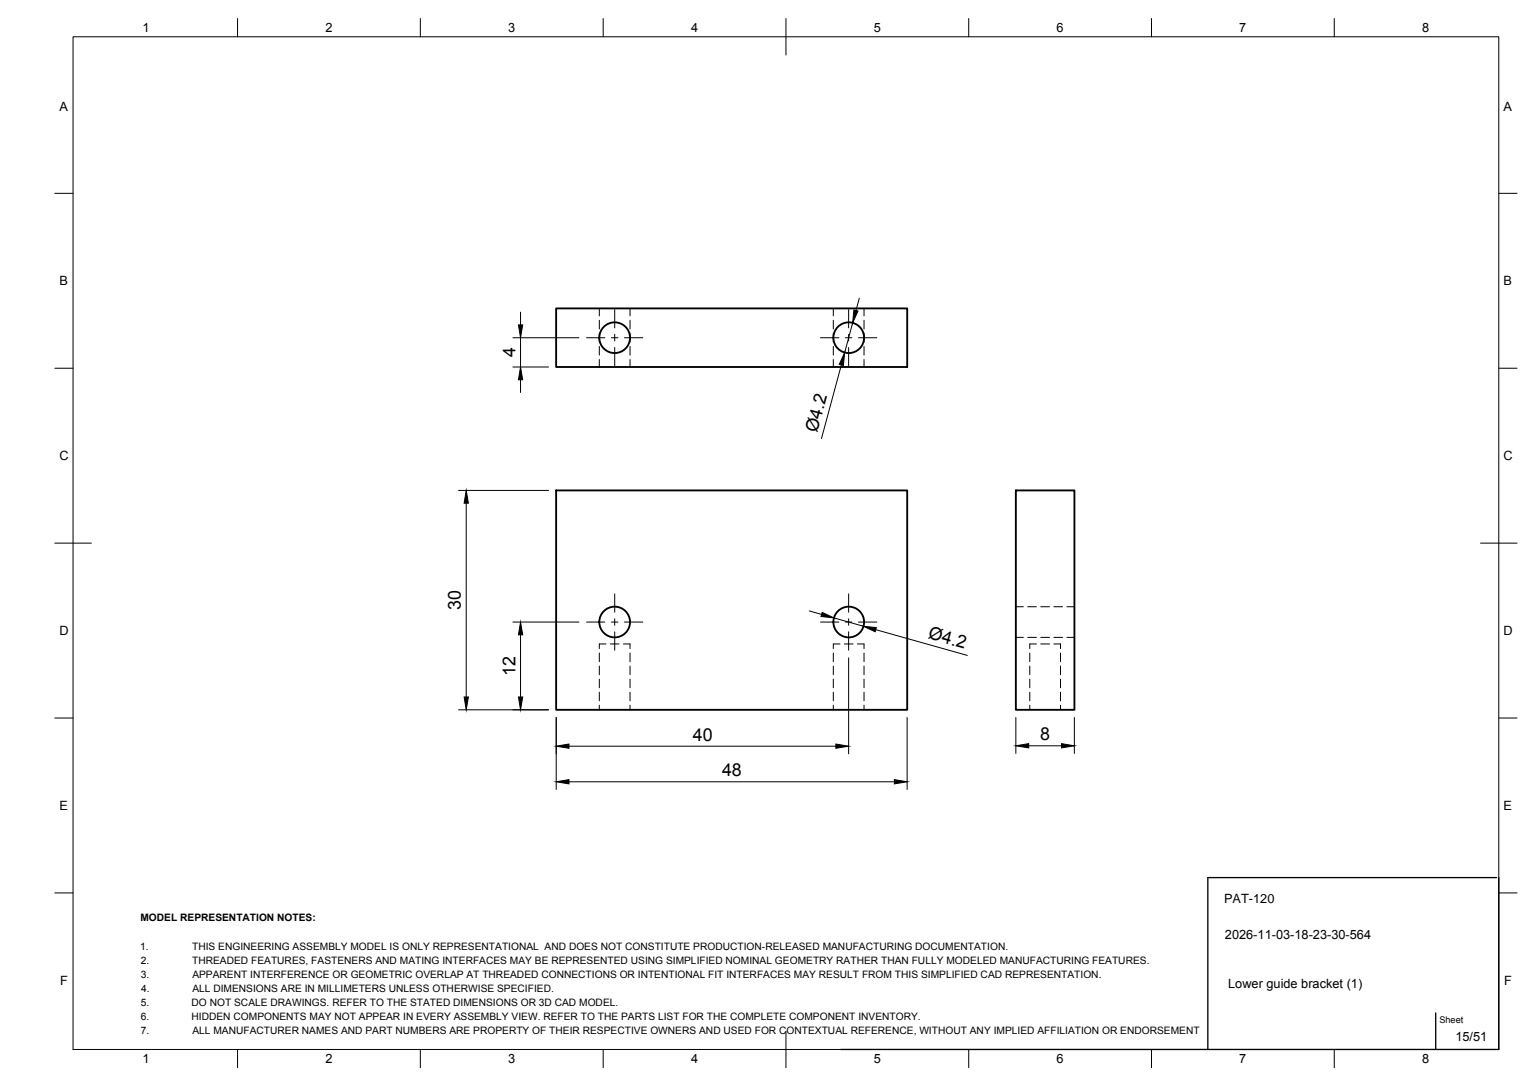
ISO-10303-21;
HEADER;
/* Generated by software containing ST-Developer
 * from STEP Tools, Inc. (www.steptools.com) 
 */

FILE_DESCRIPTION(
/* description */ ('Vibration shaker table dummy'),
/* implementation_level */ '2;1');

FILE_NAME(
/* name */ 'Lower guide bracket (1).step',
/* time_stamp */ '2026-10-27T10:55:14-07:00',
/* author */ (''),
/* organization */ (''),
/* preprocessor_version */ 'ST-DEVELOPER v20.2',
/* originating_system */ 'Autodesk Translation Framework v15.17.0.0',
/* authorisation */ '');

FILE_SCHEMA (('AUTOMOTIVE_DESIGN { 1 0 10303 214 3 1 1 }'));
ENDSEC;

DATA;
#10=MECHANICAL_DESIGN_GEOMETRIC_PRESENTATION_REPRESENTATION('',(#696),#22394);
#604=SHAPE_REPRESENTATION_RELATIONSHIP('SRR','None',#22650,#650);
#650=ADVANCED_BREP_SHAPE_REPRESENTATION('',(#742),#22356);
#696=STYLED_ITEM('',(#22940),#742);
#742=MANIFOLD_SOLID_BREP('Body1',#9214);
#877=FACE_BOUND('',#2073,.T.);
#878=FACE_BOUND('',#2074,.T.);
#879=FACE_BOUND('',#2077,.T.);
#880=FACE_BOUND('',#2078,.T.);
#881=FACE_BOUND('',#2082,.T.);
#882=FACE_BOUND('',#2083,.T.);
#1126=PLANE('',#10022);
#1127=PLANE('',#10026);
#1128=PLANE('',#10033);
#1129=PLANE('',#10034);
#1130=PLANE('',#10035);
#1131=PLANE('',#10036);
#1132=PLANE('',#10037);
#1133=PLANE('',#10038);
#1466=FACE_OUTER_BOUND('',#2066,.T.);
#1467=FACE_OUTER_BOUND('',#2067,.T.);
#1468=FACE_OUTER_BOUND('',#2068,.T.);
#1469=FACE_OUTER_BOUND('',#2069,.T.);
#1470=FACE_OUTER_BOUND('',#2070,.T.);
#1471=FACE_OUTER_BOUND('',#2071,.T.);
#1472=FACE_OUTER_BOUND('',#2072,.T.);
#1473=FACE_OUTER_BOUND('',#2075,.T.);
#1474=FACE_OUTER_BOUND('',#2076,.T.);
#1475=FACE_OUTER_BOUND('',#2079,.T.);
#1476=FACE_OUTER_BOUND('',#2080,.T.);
#1477=FACE_OUTER_BOUND('',#2081,.T.);
#2066=EDGE_LOOP('',(#6828,#6829,#6830,#6831));
#2067=EDGE_LOOP('',(#6832));
#2068=EDGE_LOOP('',(#6833,#6834,#6835,#6836));
#2069=EDGE_LOOP('',(#6837));
#2070=EDGE_LOOP('',(#6838,#6839,#6840,#6841));
#2071=EDGE_LOOP('',(#6842,#6843,#6844,#6845));
#2072=EDGE_LOOP('',(#6846,#6847,#6848,#6849));
#2073=EDGE_LOOP('',(#6850));
#2074=EDGE_LOOP('',(#6851));
#2075=EDGE_LOOP('',(#6852,#6853,#6854,#6855));
#2076=EDGE_LOOP('',(#6856,#6857,#6858,#6859));
#2077=EDGE_LOOP('',(#6860));
#2078=EDGE_LOOP('',(#6861));
#2079=EDGE_LOOP('',(#6862,#6863,#6864,#6865));
#2080=EDGE_LOOP('',(#6866,#6867,#6868,#6869));
#2081=EDGE_LOOP('',(#6870,#6871,#6872,#6873));
#2082=EDGE_LOOP('',(#6874));
#2083=EDGE_LOOP('',(#6875));
#2790=LINE('',#16048,#3409);
#2791=LINE('',#16055,#3410);
#2792=LINE('',#16062,#3411);
#2793=LINE('',#16068,#3412);
#2794=LINE('',#16073,#3413);
#2795=LINE('',#16075,#3414);
#2796=LINE('',#16077,#3415);
#2797=LINE('',#16078,#3416);
#2798=LINE('',#16081,#3417);
#2799=LINE('',#16083,#3418);
#2800=LINE('',#16084,#3419);
#2801=LINE('',#16087,#3420);
#2802=LINE('',#16089,#3421);
#2803=LINE('',#16090,#3422);
#2804=LINE('',#16092,#3423);
#2805=LINE('',#16093,#3424);
#3409=VECTOR('',#11640,0.21);
#3410=VECTOR('',#11649,0.21);
#3411=VECTOR('',#11658,0.21);
#3412=VECTOR('',#11665,0.21);
#3413=VECTOR('',#11670,1.);
#3414=VECTOR('',#11671,1.);
#3415=VECTOR('',#11672,1.);
#3416=VECTOR('',#11673,1.);
#3417=VECTOR('',#11676,1.);
#3418=VECTOR('',#11677,1.);
#3419=VECTOR('',#11678,1.);
#3420=VECTOR('',#11681,1.);
#3421=VECTOR('',#11682,1.);
#3422=VECTOR('',#11683,1.);
#3423=VECTOR('',#11686,1.);
#3424=VECTOR('',#11687,1.);
#3982=CIRCLE('',#10020,0.21);
#3983=CIRCLE('',#10021,0.21);
#3984=CIRCLE('',#10024,0.21);
#3985=CIRCLE('',#10025,0.21);
#3986=CIRCLE('',#10028,0.21);
#3987=CIRCLE('',#10029,0.21);
#3988=CIRCLE('',#10031,0.21);
#3989=CIRCLE('',#10032,0.21);
#4561=VERTEX_POINT('',#16045);
#4562=VERTEX_POINT('',#16047);
#4563=VERTEX_POINT('',#16052);
#4564=VERTEX_POINT('',#16054);
#4565=VERTEX_POINT('',#16059);
#4566=VERTEX_POINT('',#16061);
#4567=VERTEX_POINT('',#16065);
#4568=VERTEX_POINT('',#16067);
#4569=VERTEX_POINT('',#16071);
#4570=VERTEX_POINT('',#16072);
#4571=VERTEX_POINT('',#16074);
#4572=VERTEX_POINT('',#16076);
#4573=VERTEX_POINT('',#16080);
#4574=VERTEX_POINT('',#16082);
#4575=VERTEX_POINT('',#16086);
#4576=VERTEX_POINT('',#16088);
#5407=EDGE_CURVE('',#4561,#4561,#3982,.T.);
#5408=EDGE_CURVE('',#4561,#4562,#2790,.T.);
#5409=EDGE_CURVE('',#4562,#4562,#3983,.T.);
#5410=EDGE_CURVE('',#4563,#4563,#3984,.T.);
#5411=EDGE_CURVE('',#4563,#4564,#2791,.T.);
#5412=EDGE_CURVE('',#4564,#4564,#3985,.T.);
#5413=EDGE_CURVE('',#4565,#4565,#3986,.T.);
#5414=EDGE_CURVE('',#4565,#4566,#2792,.T.);
#5415=EDGE_CURVE('',#4566,#4566,#3987,.T.);
#5416=EDGE_CURVE('',#4567,#4567,#3988,.T.);
#5417=EDGE_CURVE('',#4567,#4568,#2793,.T.);
#5418=EDGE_CURVE('',#4568,#4568,#3989,.T.);
#5419=EDGE_CURVE('',#4569,#4570,#2794,.T.);
#5420=EDGE_CURVE('',#4570,#4571,#2795,.T.);
#5421=EDGE_CURVE('',#4572,#4571,#2796,.T.);
#5422=EDGE_CURVE('',#4569,#4572,#2797,.T.);
#5423=EDGE_CURVE('',#4573,#4569,#2798,.T.);
#5424=EDGE_CURVE('',#4574,#4572,#2799,.T.);
#5425=EDGE_CURVE('',#4573,#4574,#2800,.T.);
#5426=EDGE_CURVE('',#4575,#4573,#2801,.T.);
#5427=EDGE_CURVE('',#4576,#4574,#2802,.T.);
#5428=EDGE_CURVE('',#4575,#4576,#2803,.T.);
#5429=EDGE_CURVE('',#4570,#4575,#2804,.T.);
#5430=EDGE_CURVE('',#4571,#4576,#2805,.T.);
#6828=ORIENTED_EDGE('',*,*,#5407,.F.);
#6829=ORIENTED_EDGE('',*,*,#5408,.T.);
#6830=ORIENTED_EDGE('',*,*,#5409,.T.);
#6831=ORIENTED_EDGE('',*,*,#5408,.F.);
#6832=ORIENTED_EDGE('',*,*,#5409,.F.);
#6833=ORIENTED_EDGE('',*,*,#5410,.F.);
#6834=ORIENTED_EDGE('',*,*,#5411,.T.);
#6835=ORIENTED_EDGE('',*,*,#5412,.T.);
#6836=ORIENTED_EDGE('',*,*,#5411,.F.);
#6837=ORIENTED_EDGE('',*,*,#5412,.F.);
#6838=ORIENTED_EDGE('',*,*,#5413,.F.);
#6839=ORIENTED_EDGE('',*,*,#5414,.T.);
#6840=ORIENTED_EDGE('',*,*,#5415,.F.);
#6841=ORIENTED_EDGE('',*,*,#5414,.F.);
#6842=ORIENTED_EDGE('',*,*,#5416,.F.);
#6843=ORIENTED_EDGE('',*,*,#5417,.T.);
#6844=ORIENTED_EDGE('',*,*,#5418,.F.);
#6845=ORIENTED_EDGE('',*,*,#5417,.F.);
#6846=ORIENTED_EDGE('',*,*,#5419,.T.);
#6847=ORIENTED_EDGE('',*,*,#5420,.T.);
#6848=ORIENTED_EDGE('',*,*,#5421,.F.);
#6849=ORIENTED_EDGE('',*,*,#5422,.F.);
#6850=ORIENTED_EDGE('',*,*,#5415,.T.);
#6851=ORIENTED_EDGE('',*,*,#5418,.T.);
#6852=ORIENTED_EDGE('',*,*,#5423,.T.);
#6853=ORIENTED_EDGE('',*,*,#5422,.T.);
#6854=ORIENTED_EDGE('',*,*,#5424,.F.);
#6855=ORIENTED_EDGE('',*,*,#5425,.F.);
#6856=ORIENTED_EDGE('',*,*,#5426,.T.);
#6857=ORIENTED_EDGE('',*,*,#5425,.T.);
#6858=ORIENTED_EDGE('',*,*,#5427,.F.);
#6859=ORIENTED_EDGE('',*,*,#5428,.F.);
#6860=ORIENTED_EDGE('',*,*,#5413,.T.);
#6861=ORIENTED_EDGE('',*,*,#5416,.T.);
#6862=ORIENTED_EDGE('',*,*,#5429,.T.);
#6863=ORIENTED_EDGE('',*,*,#5428,.T.);
#6864=ORIENTED_EDGE('',*,*,#5430,.F.);
#6865=ORIENTED_EDGE('',*,*,#5420,.F.);
#6866=ORIENTED_EDGE('',*,*,#5430,.T.);
#6867=ORIENTED_EDGE('',*,*,#5427,.T.);
#6868=ORIENTED_EDGE('',*,*,#5424,.T.);
#6869=ORIENTED_EDGE('',*,*,#5421,.T.);
#6870=ORIENTED_EDGE('',*,*,#5429,.F.);
#6871=ORIENTED_EDGE('',*,*,#5419,.F.);
#6872=ORIENTED_EDGE('',*,*,#5423,.F.);
#6873=ORIENTED_EDGE('',*,*,#5426,.F.);
#6874=ORIENTED_EDGE('',*,*,#5407,.T.);
#6875=ORIENTED_EDGE('',*,*,#5410,.T.);
#8564=CYLINDRICAL_SURFACE('',#10019,0.21);
#8565=CYLINDRICAL_SURFACE('',#10023,0.21);
#8566=CYLINDRICAL_SURFACE('',#10027,0.21);
#8567=CYLINDRICAL_SURFACE('',#10030,0.21);
#8831=ADVANCED_FACE('',(#1466),#8564,.F.);
#8832=ADVANCED_FACE('',(#1467),#1126,.F.);
#8833=ADVANCED_FACE('',(#1468),#8565,.F.);
#8834=ADVANCED_FACE('',(#1469),#1127,.F.);
#8835=ADVANCED_FACE('',(#1470),#8566,.F.);
#8836=ADVANCED_FACE('',(#1471),#8567,.F.);
#8837=ADVANCED_FACE('',(#1472,#877,#878),#1128,.T.);
#8838=ADVANCED_FACE('',(#1473),#1129,.T.);
#8839=ADVANCED_FACE('',(#1474,#879,#880),#1130,.T.);
#8840=ADVANCED_FACE('',(#1475),#1131,.T.);
#8841=ADVANCED_FACE('',(#1476),#1132,.T.);
#8842=ADVANCED_FACE('',(#1477,#881,#882),#1133,.F.);
#9214=CLOSED_SHELL('',(#8831,#8832,#8833,#8834,#8835,#8836,#8837,#8838,
#8839,#8840,#8841,#8842));
#10018=AXIS2_PLACEMENT_3D('',#16043,#11634,#11635);
#10019=AXIS2_PLACEMENT_3D('',#16044,#11636,#11637);
#10020=AXIS2_PLACEMENT_3D('',#16046,#11638,#11639);
#10021=AXIS2_PLACEMENT_3D('',#16049,#11641,#11642);
#10022=AXIS2_PLACEMENT_3D('',#16050,#11643,#11644);
#10023=AXIS2_PLACEMENT_3D('',#16051,#11645,#11646);
#10024=AXIS2_PLACEMENT_3D('',#16053,#11647,#11648);
#10025=AXIS2_PLACEMENT_3D('',#16056,#11650,#11651);
#10026=AXIS2_PLACEMENT_3D('',#16057,#11652,#11653);
#10027=AXIS2_PLACEMENT_3D('',#16058,#11654,#11655);
#10028=AXIS2_PLACEMENT_3D('',#16060,#11656,#11657);
#10029=AXIS2_PLACEMENT_3D('',#16063,#11659,#11660);
#10030=AXIS2_PLACEMENT_3D('',#16064,#11661,#11662);
#10031=AXIS2_PLACEMENT_3D('',#16066,#11663,#11664);
#10032=AXIS2_PLACEMENT_3D('',#16069,#11666,#11667);
#10033=AXIS2_PLACEMENT_3D('',#16070,#11668,#11669);
#10034=AXIS2_PLACEMENT_3D('',#16079,#11674,#11675);
#10035=AXIS2_PLACEMENT_3D('',#16085,#11679,#11680);
#10036=AXIS2_PLACEMENT_3D('',#16091,#11684,#11685);
#10037=AXIS2_PLACEMENT_3D('',#16094,#11688,#11689);
#10038=AXIS2_PLACEMENT_3D('',#16095,#11690,#11691);
#11634=DIRECTION('axis',(0.,0.,1.));
#11635=DIRECTION('refdir',(1.,0.,0.));
#11636=DIRECTION('center_axis',(0.,0.,1.));
#11637=DIRECTION('ref_axis',(1.,0.,0.));
#11638=DIRECTION('center_axis',(0.,0.,1.));
#11639=DIRECTION('ref_axis',(1.,0.,0.));
#11640=DIRECTION('',(0.,0.,1.));
#11641=DIRECTION('center_axis',(0.,0.,1.));
#11642=DIRECTION('ref_axis',(1.,0.,0.));
#11643=DIRECTION('center_axis',(0.,0.,1.));
#11644=DIRECTION('ref_axis',(1.,0.,0.));
#11645=DIRECTION('center_axis',(0.,0.,1.));
#11646=DIRECTION('ref_axis',(1.,0.,0.));
#11647=DIRECTION('center_axis',(0.,0.,1.));
#11648=DIRECTION('ref_axis',(1.,0.,0.));
#11649=DIRECTION('',(0.,0.,1.));
#11650=DIRECTION('center_axis',(0.,0.,1.));
#11651=DIRECTION('ref_axis',(1.,0.,0.));
#11652=DIRECTION('center_axis',(0.,0.,1.));
#11653=DIRECTION('ref_axis',(1.,0.,0.));
#11654=DIRECTION('center_axis',(0.,1.,0.));
#11655=DIRECTION('ref_axis',(1.,0.,0.));
#11656=DIRECTION('center_axis',(0.,1.,0.));
#11657=DIRECTION('ref_axis',(1.,0.,0.));
#11658=DIRECTION('',(0.,1.,0.));
#11659=DIRECTION('center_axis',(0.,-1.,0.));
#11660=DIRECTION('ref_axis',(1.,0.,0.));
#11661=DIRECTION('center_axis',(0.,1.,0.));
#11662=DIRECTION('ref_axis',(1.,0.,0.));
#11663=DIRECTION('center_axis',(0.,1.,0.));
#11664=DIRECTION('ref_axis',(1.,0.,0.));
#11665=DIRECTION('',(0.,1.,0.));
#11666=DIRECTION('center_axis',(0.,-1.,0.));
#11667=DIRECTION('ref_axis',(1.,0.,0.));
#11668=DIRECTION('center_axis',(0.,1.,0.));
#11669=DIRECTION('ref_axis',(-1.,0.,0.));
#11670=DIRECTION('',(-1.,0.,0.));
#11671=DIRECTION('',(0.,0.,1.));
#11672=DIRECTION('',(-1.,0.,0.));
#11673=DIRECTION('',(0.,0.,1.));
#11674=DIRECTION('center_axis',(1.,0.,0.));
#11675=DIRECTION('ref_axis',(0.,1.,0.));
#11676=DIRECTION('',(0.,1.,0.));
#11677=DIRECTION('',(0.,1.,0.));
#11678=DIRECTION('',(0.,0.,1.));
#11679=DIRECTION('center_axis',(0.,-1.,0.));
#11680=DIRECTION('ref_axis',(1.,0.,0.));
#11681=DIRECTION('',(1.,0.,0.));
#11682=DIRECTION('',(1.,0.,0.));
#11683=DIRECTION('',(0.,0.,1.));
#11684=DIRECTION('center_axis',(-1.,0.,0.));
#11685=DIRECTION('ref_axis',(0.,-1.,0.));
#11686=DIRECTION('',(0.,-1.,0.));
#11687=DIRECTION('',(0.,-1.,0.));
#11688=DIRECTION('center_axis',(0.,0.,1.));
#11689=DIRECTION('ref_axis',(1.,0.,0.));
#11690=DIRECTION('center_axis',(0.,0.,1.));
#11691=DIRECTION('ref_axis',(1.,0.,0.));
#16043=CARTESIAN_POINT('',(0.,0.,0.));
#16044=CARTESIAN_POINT('Origin',(-7.6,6.7,-0.1));
#16045=CARTESIAN_POINT('',(-7.81,6.7,0.));
#16046=CARTESIAN_POINT('Origin',(-7.6,6.7,0.));
#16047=CARTESIAN_POINT('',(-7.81,6.7,0.9));
#16048=CARTESIAN_POINT('',(-7.81,6.7,-0.1));
#16049=CARTESIAN_POINT('Origin',(-7.6,6.7,0.9));
#16050=CARTESIAN_POINT('Origin',(-7.6,6.7,0.9));
#16051=CARTESIAN_POINT('Origin',(-4.4,6.7,-0.1));
#16052=CARTESIAN_POINT('',(-4.61,6.7,0.));
#16053=CARTESIAN_POINT('Origin',(-4.4,6.7,0.));
#16054=CARTESIAN_POINT('',(-4.61,6.7,0.9));
#16055=CARTESIAN_POINT('',(-4.61,6.7,-0.1));
#16056=CARTESIAN_POINT('Origin',(-4.4,6.7,0.9));
#16057=CARTESIAN_POINT('Origin',(-4.4,6.7,0.9));
#16058=CARTESIAN_POINT('Origin',(-7.6,6.2,1.2));
#16059=CARTESIAN_POINT('',(-7.81,6.3,1.2));
#16060=CARTESIAN_POINT('Origin',(-7.6,6.3,1.2));
#16061=CARTESIAN_POINT('',(-7.81,7.1,1.2));
#16062=CARTESIAN_POINT('',(-7.81,6.2,1.2));
#16063=CARTESIAN_POINT('Origin',(-7.6,7.1,1.2));
#16064=CARTESIAN_POINT('Origin',(-4.4,6.2,1.2));
#16065=CARTESIAN_POINT('',(-4.61,6.3,1.2));
#16066=CARTESIAN_POINT('Origin',(-4.4,6.3,1.2));
#16067=CARTESIAN_POINT('',(-4.61,7.1,1.2));
#16068=CARTESIAN_POINT('',(-4.61,6.2,1.2));
#16069=CARTESIAN_POINT('Origin',(-4.4,7.1,1.2));
#16070=CARTESIAN_POINT('Origin',(-3.6,7.1,0.));
#16071=CARTESIAN_POINT('',(-3.6,7.1,0.));
#16072=CARTESIAN_POINT('',(-8.4,7.1,0.));
#16073=CARTESIAN_POINT('',(-3.6,7.1,0.));
#16074=CARTESIAN_POINT('',(-8.4,7.1,3.));
#16075=CARTESIAN_POINT('',(-8.4,7.1,0.));
#16076=CARTESIAN_POINT('',(-3.6,7.1,3.));
#16077=CARTESIAN_POINT('',(-3.6,7.1,3.));
#16078=CARTESIAN_POINT('',(-3.6,7.1,0.));
#16079=CARTESIAN_POINT('Origin',(-3.6,6.3,0.));
#16080=CARTESIAN_POINT('',(-3.6,6.3,0.));
#16081=CARTESIAN_POINT('',(-3.6,6.3,0.));
#16082=CARTESIAN_POINT('',(-3.6,6.3,3.));
#16083=CARTESIAN_POINT('',(-3.6,6.3,3.));
#16084=CARTESIAN_POINT('',(-3.6,6.3,0.));
#16085=CARTESIAN_POINT('Origin',(-8.4,6.3,0.));
#16086=CARTESIAN_POINT('',(-8.4,6.3,0.));
#16087=CARTESIAN_POINT('',(-8.4,6.3,0.));
#16088=CARTESIAN_POINT('',(-8.4,6.3,3.));
#16089=CARTESIAN_POINT('',(-8.4,6.3,3.));
#16090=CARTESIAN_POINT('',(-8.4,6.3,0.));
#16091=CARTESIAN_POINT('Origin',(-8.4,7.1,0.));
#16092=CARTESIAN_POINT('',(-8.4,7.1,0.));
#16093=CARTESIAN_POINT('',(-8.4,7.1,3.));
#16094=CARTESIAN_POINT('Origin',(-6.,6.7,3.));
#16095=CARTESIAN_POINT('Origin',(-6.,6.7,0.));
#22305=UNCERTAINTY_MEASURE_WITH_UNIT(LENGTH_MEASURE(0.001),#22395,
'DISTANCE_ACCURACY_VALUE',
'Maximum model space distance between geometric entities at asserted c
onnectivities');
#22343=UNCERTAINTY_MEASURE_WITH_UNIT(LENGTH_MEASURE(0.001),#22395,
'DISTANCE_ACCURACY_VALUE',
'Maximum model space distance between geometric entities at asserted c
onnectivities');
#22356=(
GEOMETRIC_REPRESENTATION_CONTEXT(3)
GLOBAL_UNCERTAINTY_ASSIGNED_CONTEXT((#22305))
GLOBAL_UNIT_ASSIGNED_CONTEXT((#22395,#22397,#22398))
REPRESENTATION_CONTEXT('','3D')
);
#22394=(
GEOMETRIC_REPRESENTATION_CONTEXT(3)
GLOBAL_UNCERTAINTY_ASSIGNED_CONTEXT((#22343))
GLOBAL_UNIT_ASSIGNED_CONTEXT((#22395,#22397,#22398))
REPRESENTATION_CONTEXT('','3D')
);
#22395=(
LENGTH_UNIT()
NAMED_UNIT(*)
SI_UNIT(.CENTI.,.METRE.)
);
#22397=(
NAMED_UNIT(*)
PLANE_ANGLE_UNIT()
SI_UNIT($,.RADIAN.)
);
#22398=(
NAMED_UNIT(*)
SI_UNIT($,.STERADIAN.)
SOLID_ANGLE_UNIT()
);
#22411=SHAPE_DEFINITION_REPRESENTATION(#22461,#22650);
#22461=PRODUCT_DEFINITION_SHAPE('',$,#22701);
#22650=SHAPE_REPRESENTATION('',(#10018),#22356);
#22688=PRODUCT_DEFINITION_CONTEXT('part definition',#22840,'design');
#22701=PRODUCT_DEFINITION('Lower guide bracket (1)',
'Lower guide bracket (1)',#22751,#22688);
#22751=PRODUCT_DEFINITION_FORMATION('',$,#22854);
#22840=APPLICATION_CONTEXT(
'Core Data for Automotive Mechanical Design Process');
#22841=PRODUCT_CONTEXT('part definition',#22840,'mechanical');
#22854=PRODUCT('Lower guide bracket (1)','Lower guide bracket (1)',
'Lower guide bracket (1)',(#22841));
#22934=COLOUR_RGB('Dark Blue',0.08,0.2,0.34);
#22935=FILL_AREA_STYLE_COLOUR('',#22934);
#22936=FILL_AREA_STYLE('',(#22935));
#22937=SURFACE_STYLE_FILL_AREA(#22936);
#22938=SURFACE_SIDE_STYLE('',(#22937));
#22939=SURFACE_STYLE_USAGE(.BOTH.,#22938);
#22940=PRESENTATION_STYLE_ASSIGNMENT((#22939));
ENDSEC;
END-ISO-10303-21;
